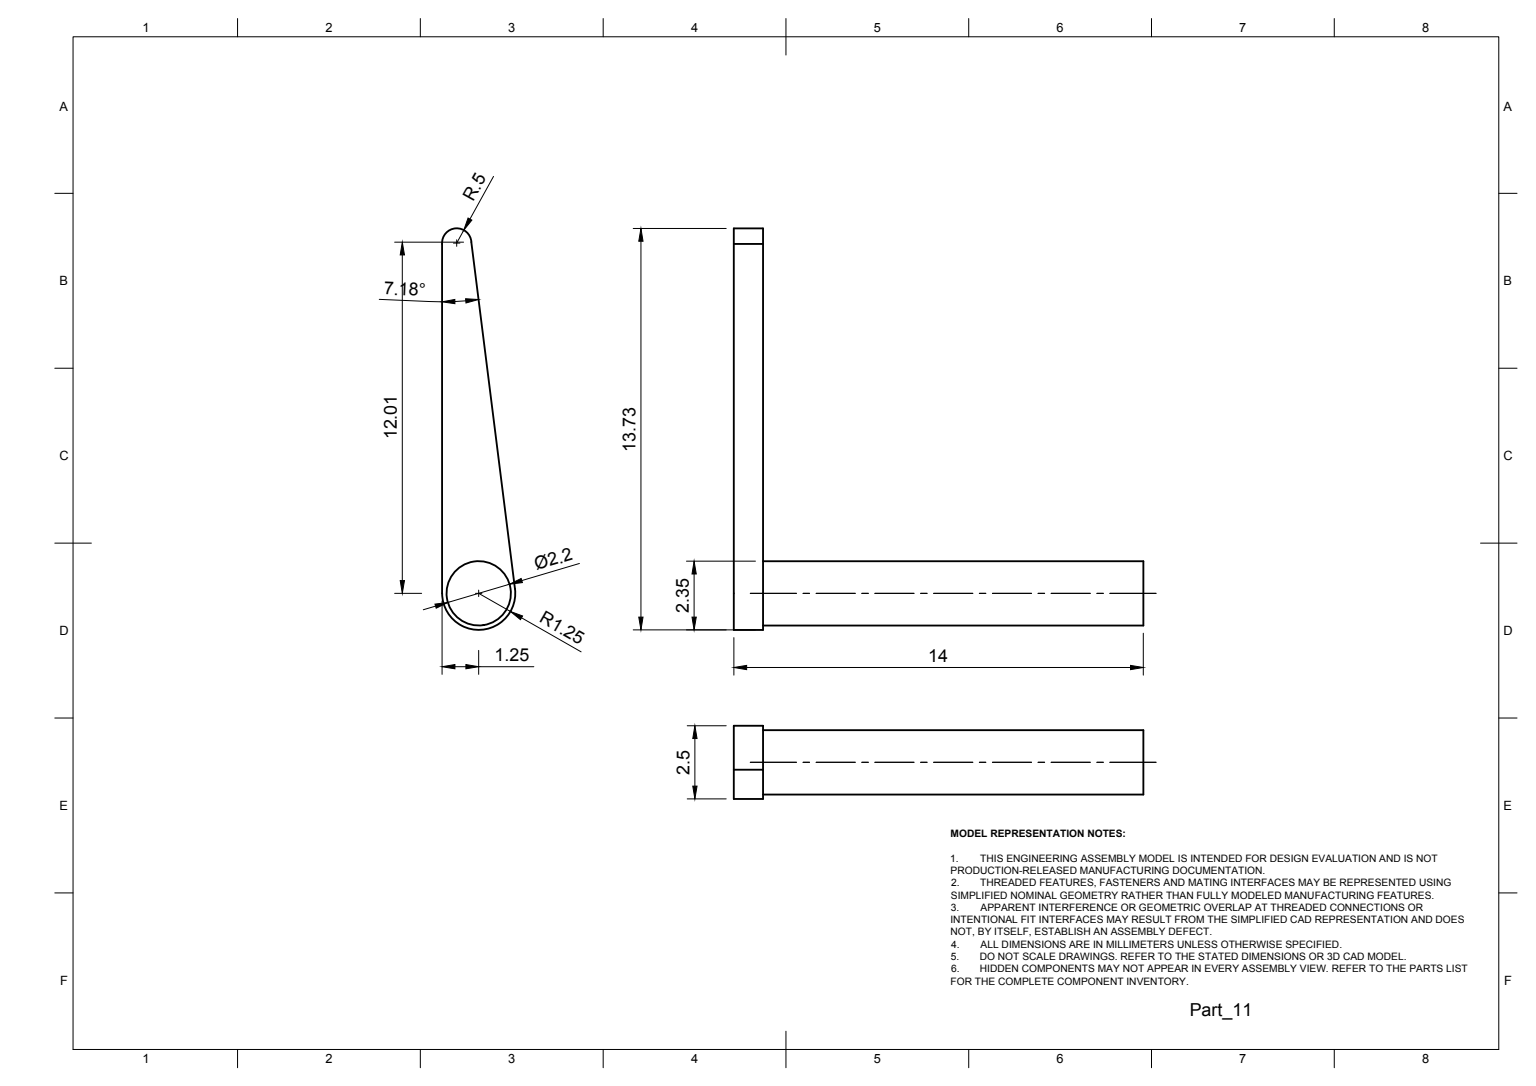
ISO-10303-21;
HEADER;
/* Generated by software containing ST-Developer
 * from STEP Tools, Inc. (www.steptools.com) 
 */

FILE_DESCRIPTION(
/* description */ ('STEP AP242 Edition 2'),
/* implementation_level */ '2;1');

FILE_NAME(
/* name */ 'Part_11.step',
/* time_stamp */ '2026-10-06T10:11:12-07:00',
/* author */ (''),
/* organization */ (''),
/* preprocessor_version */ 'ST-DEVELOPER v20.2',
/* originating_system */ 'Autodesk Translation Framework v15.15.0.0',
/* authorisation */ '');

FILE_SCHEMA (('AUTOMOTIVE_DESIGN { 1 0 10303 214 3 1 1 }'));
ENDSEC;

DATA;
#10=MECHANICAL_DESIGN_GEOMETRIC_PRESENTATION_REPRESENTATION('',(#1794),#54580);
#1750=SHAPE_REPRESENTATION_RELATIONSHIP('SRR','None',#54637,#1764);
#1764=ADVANCED_BREP_SHAPE_REPRESENTATION('',(#1808),#54573);
#1794=STYLED_ITEM('',(#54712),#1808);
#1808=MANIFOLD_SOLID_BREP('Body1',#17673);
#2251=LINE('',#48527,#2844);
#2252=LINE('',#48535,#2845);
#2253=LINE('',#48538,#2846);
#2254=LINE('',#48541,#2847);
#2255=LINE('',#48543,#2848);
#2256=LINE('',#48544,#2849);
#2257=LINE('',#48549,#2850);
#2258=LINE('',#48552,#2851);
#2259=LINE('',#48553,#2852);
#2844=VECTOR('',#22469,0.0011);
#2845=VECTOR('',#22478,1.);
#2846=VECTOR('',#22481,1.);
#2847=VECTOR('',#22484,1.);
#2848=VECTOR('',#22485,1.);
#2849=VECTOR('',#22486,1.);
#2850=VECTOR('',#22491,1.);
#2851=VECTOR('',#22496,1.);
#2852=VECTOR('',#22497,1.);
#3395=CYLINDRICAL_SURFACE('',#19049,0.0011);
#3396=CYLINDRICAL_SURFACE('',#19053,0.0005);
#3397=CYLINDRICAL_SURFACE('',#19057,0.00125);
#3510=FACE_BOUND('',#5333,.T.);
#4287=FACE_OUTER_BOUND('',#5326,.T.);
#4288=FACE_OUTER_BOUND('',#5327,.T.);
#4289=FACE_OUTER_BOUND('',#5328,.T.);
#4290=FACE_OUTER_BOUND('',#5329,.T.);
#4291=FACE_OUTER_BOUND('',#5330,.T.);
#4292=FACE_OUTER_BOUND('',#5331,.T.);
#4293=FACE_OUTER_BOUND('',#5332,.T.);
#4294=FACE_OUTER_BOUND('',#5334,.T.);
#5326=EDGE_LOOP('',(#15273,#15274,#15275,#15276));
#5327=EDGE_LOOP('',(#15277));
#5328=EDGE_LOOP('',(#15278,#15279,#15280,#15281));
#5329=EDGE_LOOP('',(#15282,#15283,#15284,#15285));
#5330=EDGE_LOOP('',(#15286,#15287,#15288,#15289));
#5331=EDGE_LOOP('',(#15290,#15291,#15292,#15293));
#5332=EDGE_LOOP('',(#15294,#15295,#15296,#15297));
#5333=EDGE_LOOP('',(#15298));
#5334=EDGE_LOOP('',(#15299,#15300,#15301,#15302));
#6227=CIRCLE('',#19050,0.0011);
#6228=CIRCLE('',#19051,0.0011);
#6229=CIRCLE('',#19054,0.0005);
#6230=CIRCLE('',#19055,0.0005);
#6231=CIRCLE('',#19058,0.00125);
#6232=CIRCLE('',#19059,0.00125);
#7924=VERTEX_POINT('',#48524);
#7925=VERTEX_POINT('',#48526);
#7926=VERTEX_POINT('',#48531);
#7927=VERTEX_POINT('',#48532);
#7928=VERTEX_POINT('',#48534);
#7929=VERTEX_POINT('',#48536);
#7930=VERTEX_POINT('',#48540);
#7931=VERTEX_POINT('',#48542);
#7932=VERTEX_POINT('',#48546);
#7933=VERTEX_POINT('',#48548);
#10428=EDGE_CURVE('',#7924,#7924,#6227,.F.);
#10429=EDGE_CURVE('',#7924,#7925,#2251,.T.);
#10430=EDGE_CURVE('',#7925,#7925,#6228,.F.);
#10431=EDGE_CURVE('',#7926,#7927,#6229,.T.);
#10432=EDGE_CURVE('',#7928,#7926,#2252,.T.);
#10433=EDGE_CURVE('',#7928,#7929,#6230,.T.);
#10434=EDGE_CURVE('',#7929,#7927,#2253,.T.);
#10435=EDGE_CURVE('',#7930,#7926,#2254,.T.);
#10436=EDGE_CURVE('',#7931,#7930,#2255,.T.);
#10437=EDGE_CURVE('',#7931,#7928,#2256,.T.);
#10438=EDGE_CURVE('',#7932,#7930,#6231,.T.);
#10439=EDGE_CURVE('',#7933,#7932,#2257,.T.);
#10440=EDGE_CURVE('',#7933,#7931,#6232,.T.);
#10441=EDGE_CURVE('',#7927,#7932,#2258,.T.);
#10442=EDGE_CURVE('',#7929,#7933,#2259,.T.);
#15273=ORIENTED_EDGE('',*,*,#10428,.T.);
#15274=ORIENTED_EDGE('',*,*,#10429,.T.);
#15275=ORIENTED_EDGE('',*,*,#10430,.T.);
#15276=ORIENTED_EDGE('',*,*,#10429,.F.);
#15277=ORIENTED_EDGE('',*,*,#10430,.F.);
#15278=ORIENTED_EDGE('',*,*,#10431,.F.);
#15279=ORIENTED_EDGE('',*,*,#10432,.F.);
#15280=ORIENTED_EDGE('',*,*,#10433,.T.);
#15281=ORIENTED_EDGE('',*,*,#10434,.T.);
#15282=ORIENTED_EDGE('',*,*,#10435,.F.);
#15283=ORIENTED_EDGE('',*,*,#10436,.F.);
#15284=ORIENTED_EDGE('',*,*,#10437,.T.);
#15285=ORIENTED_EDGE('',*,*,#10432,.T.);
#15286=ORIENTED_EDGE('',*,*,#10438,.F.);
#15287=ORIENTED_EDGE('',*,*,#10439,.F.);
#15288=ORIENTED_EDGE('',*,*,#10440,.T.);
#15289=ORIENTED_EDGE('',*,*,#10436,.T.);
#15290=ORIENTED_EDGE('',*,*,#10441,.F.);
#15291=ORIENTED_EDGE('',*,*,#10434,.F.);
#15292=ORIENTED_EDGE('',*,*,#10442,.T.);
#15293=ORIENTED_EDGE('',*,*,#10439,.T.);
#15294=ORIENTED_EDGE('',*,*,#10433,.F.);
#15295=ORIENTED_EDGE('',*,*,#10437,.F.);
#15296=ORIENTED_EDGE('',*,*,#10440,.F.);
#15297=ORIENTED_EDGE('',*,*,#10442,.F.);
#15298=ORIENTED_EDGE('',*,*,#10428,.F.);
#15299=ORIENTED_EDGE('',*,*,#10431,.T.);
#15300=ORIENTED_EDGE('',*,*,#10441,.T.);
#15301=ORIENTED_EDGE('',*,*,#10438,.T.);
#15302=ORIENTED_EDGE('',*,*,#10435,.T.);
#16607=PLANE('',#19052);
#16608=PLANE('',#19056);
#16609=PLANE('',#19060);
#16610=PLANE('',#19061);
#16611=PLANE('',#19062);
#17403=ADVANCED_FACE('',(#4287),#3395,.T.);
#17404=ADVANCED_FACE('',(#4288),#16607,.T.);
#17405=ADVANCED_FACE('',(#4289),#3396,.T.);
#17406=ADVANCED_FACE('',(#4290),#16608,.T.);
#17407=ADVANCED_FACE('',(#4291),#3397,.T.);
#17408=ADVANCED_FACE('',(#4292),#16609,.T.);
#17409=ADVANCED_FACE('',(#4293,#3510),#16610,.F.);
#17410=ADVANCED_FACE('',(#4294),#16611,.T.);
#17673=CLOSED_SHELL('',(#17403,#17404,#17405,#17406,#17407,#17408,#17409,
#17410));
#19048=AXIS2_PLACEMENT_3D('',#48522,#22463,#22464);
#19049=AXIS2_PLACEMENT_3D('',#48523,#22465,#22466);
#19050=AXIS2_PLACEMENT_3D('',#48525,#22467,#22468);
#19051=AXIS2_PLACEMENT_3D('',#48528,#22470,#22471);
#19052=AXIS2_PLACEMENT_3D('',#48529,#22472,#22473);
#19053=AXIS2_PLACEMENT_3D('',#48530,#22474,#22475);
#19054=AXIS2_PLACEMENT_3D('',#48533,#22476,#22477);
#19055=AXIS2_PLACEMENT_3D('',#48537,#22479,#22480);
#19056=AXIS2_PLACEMENT_3D('',#48539,#22482,#22483);
#19057=AXIS2_PLACEMENT_3D('',#48545,#22487,#22488);
#19058=AXIS2_PLACEMENT_3D('',#48547,#22489,#22490);
#19059=AXIS2_PLACEMENT_3D('',#48550,#22492,#22493);
#19060=AXIS2_PLACEMENT_3D('',#48551,#22494,#22495);
#19061=AXIS2_PLACEMENT_3D('',#48554,#22498,#22499);
#19062=AXIS2_PLACEMENT_3D('',#48555,#22500,#22501);
#22463=DIRECTION('axis',(0.,0.,1.));
#22464=DIRECTION('refdir',(1.,0.,0.));
#22465=DIRECTION('center_axis',(0.,1.,0.));
#22466=DIRECTION('ref_axis',(0.,0.,1.));
#22467=DIRECTION('center_axis',(0.,1.,0.));
#22468=DIRECTION('ref_axis',(0.,0.,1.));
#22469=DIRECTION('',(0.,-1.,0.));
#22470=DIRECTION('center_axis',(0.,-1.,0.));
#22471=DIRECTION('ref_axis',(0.,0.,-1.));
#22472=DIRECTION('center_axis',(0.,-1.,0.));
#22473=DIRECTION('ref_axis',(0.,0.,-1.));
#22474=DIRECTION('center_axis',(0.,1.,0.));
#22475=DIRECTION('ref_axis',(1.22464679914735E-16,0.,-1.));
#22476=DIRECTION('center_axis',(0.,1.,0.));
#22477=DIRECTION('ref_axis',(0.,0.,1.));
#22478=DIRECTION('',(0.,1.,0.));
#22479=DIRECTION('center_axis',(0.,1.,0.));
#22480=DIRECTION('ref_axis',(0.,0.,1.));
#22481=DIRECTION('',(0.,1.,0.));
#22482=DIRECTION('center_axis',(0.998039845995171,0.,-0.0625816730835345));
#22483=DIRECTION('ref_axis',(-0.0625816730835345,0.,-0.998039845995171));
#22484=DIRECTION('',(-0.0625816730835345,0.,-0.998039845995171));
#22485=DIRECTION('',(0.,1.,0.));
#22486=DIRECTION('',(-0.0625816730835345,0.,-0.998039845995171));
#22487=DIRECTION('center_axis',(0.,1.,0.));
#22488=DIRECTION('ref_axis',(0.,0.,1.));
#22489=DIRECTION('center_axis',(0.,1.,0.));
#22490=DIRECTION('ref_axis',(0.,0.,1.));
#22491=DIRECTION('',(0.,1.,0.));
#22492=DIRECTION('center_axis',(0.,1.,0.));
#22493=DIRECTION('ref_axis',(0.,0.,1.));
#22494=DIRECTION('center_axis',(-0.998039845995171,0.,-0.0625816730835345));
#22495=DIRECTION('ref_axis',(-0.0625816730835345,0.,0.998039845995171));
#22496=DIRECTION('',(-0.0625816730835345,0.,0.998039845995171));
#22497=DIRECTION('',(-0.0625816730835345,0.,0.998039845995171));
#22498=DIRECTION('center_axis',(0.,1.,0.));
#22499=DIRECTION('ref_axis',(0.,0.,1.));
#22500=DIRECTION('center_axis',(0.,1.,0.));
#22501=DIRECTION('ref_axis',(0.,0.,1.));
#48522=CARTESIAN_POINT('',(0.,0.,0.));
#48523=CARTESIAN_POINT('Origin',(0.,-0.00311126983722081,0.));
#48524=CARTESIAN_POINT('',(-1.34711147906209E-19,0.013,-0.0011));
#48525=CARTESIAN_POINT('Origin',(0.,0.013,0.));
#48526=CARTESIAN_POINT('',(0.,0.,-0.0011));
#48527=CARTESIAN_POINT('',(-1.34711147906209E-19,-0.00311126983722081,-0.0011));
#48528=CARTESIAN_POINT('Origin',(0.,0.,0.));
#48529=CARTESIAN_POINT('Origin',(0.00213706124849222,0.,0.000772521431045073));
#48530=CARTESIAN_POINT('Origin',(0.,0.013,-0.012));
#48531=CARTESIAN_POINT('',(0.0005,0.014,-0.012));
#48532=CARTESIAN_POINT('',(-0.0005,0.014,-0.012));
#48533=CARTESIAN_POINT('Origin',(0.,0.014,-0.012));
#48534=CARTESIAN_POINT('',(0.0005,0.013,-0.012));
#48535=CARTESIAN_POINT('',(0.0005,0.013,-0.012));
#48536=CARTESIAN_POINT('',(-0.0005,0.013,-0.012));
#48537=CARTESIAN_POINT('Origin',(0.,0.013,-0.012));
#48538=CARTESIAN_POINT('',(-0.0005,0.013,-0.012));
#48539=CARTESIAN_POINT('Origin',(0.0005,0.013,-0.012));
#48540=CARTESIAN_POINT('',(0.00124754980749396,0.014,-7.8227091354418E-5));
#48541=CARTESIAN_POINT('',(0.0005,0.014,-0.012));
#48542=CARTESIAN_POINT('',(0.00124754980749396,0.013,-7.8227091354418E-5));
#48543=CARTESIAN_POINT('',(0.00124754980749396,0.013,-7.8227091354418E-5));
#48544=CARTESIAN_POINT('',(0.0005,0.013,-0.012));
#48545=CARTESIAN_POINT('Origin',(0.,0.013,0.));
#48546=CARTESIAN_POINT('',(-0.00124754980749396,0.014,-7.82270913544182E-5));
#48547=CARTESIAN_POINT('Origin',(0.,0.014,0.));
#48548=CARTESIAN_POINT('',(-0.00124754980749396,0.013,-7.82270913544182E-5));
#48549=CARTESIAN_POINT('',(-0.00124754980749396,0.013,-7.82270913544182E-5));
#48550=CARTESIAN_POINT('Origin',(0.,0.013,0.));
#48551=CARTESIAN_POINT('Origin',(-0.0005,0.013,-0.012));
#48552=CARTESIAN_POINT('',(-0.0005,0.014,-0.012));
#48553=CARTESIAN_POINT('',(-0.0005,0.013,-0.012));
#48554=CARTESIAN_POINT('Origin',(0.,0.013,-0.012));
#48555=CARTESIAN_POINT('Origin',(0.,0.014,0.));
#54557=UNCERTAINTY_MEASURE_WITH_UNIT(LENGTH_MEASURE(1.E-5),#54581,
'DISTANCE_ACCURACY_VALUE',
'Maximum model space distance between geometric entities at asserted c
onnectivities');
#54564=UNCERTAINTY_MEASURE_WITH_UNIT(LENGTH_MEASURE(1.E-5),#54581,
'DISTANCE_ACCURACY_VALUE',
'Maximum model space distance between geometric entities at asserted c
onnectivities');
#54573=(
GEOMETRIC_REPRESENTATION_CONTEXT(3)
GLOBAL_UNCERTAINTY_ASSIGNED_CONTEXT((#54557))
GLOBAL_UNIT_ASSIGNED_CONTEXT((#54581,#54582,#54583))
REPRESENTATION_CONTEXT('','3D')
);
#54580=(
GEOMETRIC_REPRESENTATION_CONTEXT(3)
GLOBAL_UNCERTAINTY_ASSIGNED_CONTEXT((#54564))
GLOBAL_UNIT_ASSIGNED_CONTEXT((#54581,#54582,#54583))
REPRESENTATION_CONTEXT('','3D')
);
#54581=(
LENGTH_UNIT()
NAMED_UNIT(*)
SI_UNIT($,.METRE.)
);
#54582=(
NAMED_UNIT(*)
PLANE_ANGLE_UNIT()
SI_UNIT($,.RADIAN.)
);
#54583=(
NAMED_UNIT(*)
SI_UNIT($,.STERADIAN.)
SOLID_ANGLE_UNIT()
);
#54592=SHAPE_DEFINITION_REPRESENTATION(#54607,#54637);
#54607=PRODUCT_DEFINITION_SHAPE('',$,#54653);
#54637=SHAPE_REPRESENTATION('',(#19048),#54573);
#54644=PRODUCT_DEFINITION_CONTEXT('part definition',#54691,'design');
#54653=PRODUCT_DEFINITION('Part_11','Part_11',#54668,#54644);
#54668=PRODUCT_DEFINITION_FORMATION('',$,#54701);
#54691=APPLICATION_CONTEXT(
'Core Data for Automotive Mechanical Design Process');
#54692=PRODUCT_CONTEXT('part definition',#54691,'mechanical');
#54701=PRODUCT('Part_11','Part_11','Part 1',(#54692));
#54712=PRESENTATION_STYLE_ASSIGNMENT((#54722));
#54722=SURFACE_STYLE_USAGE(.BOTH.,#54732);
#54732=SURFACE_SIDE_STYLE('',(#54742));
#54742=SURFACE_STYLE_FILL_AREA(#54752);
#54752=FILL_AREA_STYLE('Opaque(26,26,26)',(#54762));
#54762=FILL_AREA_STYLE_COLOUR('Opaque(26,26,26)',#54772);
#54772=COLOUR_RGB('Opaque(26,26,26)', 0.66274510, 0.83137255, 0.94901961);
ENDSEC;
END-ISO-10303-21;
